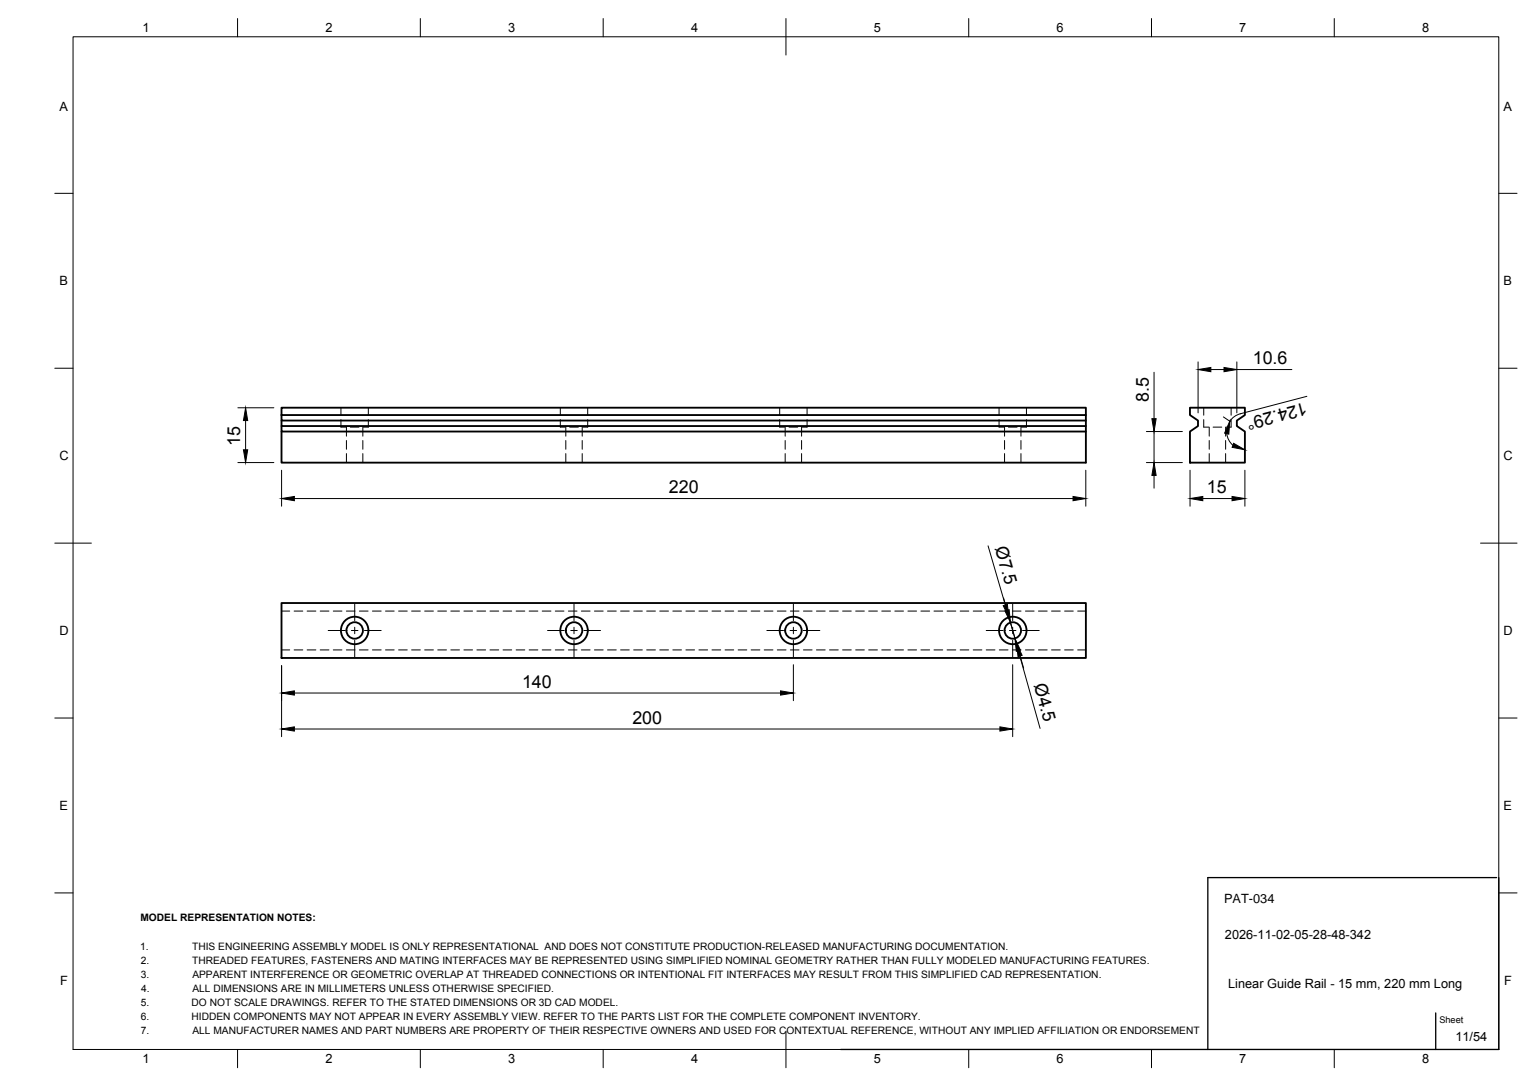
ISO-10303-21;
HEADER;
/* Generated by software containing ST-Developer
 * from STEP Tools, Inc. (www.steptools.com) 
 */

FILE_DESCRIPTION(
/* description */ ('Fatigue rig crank-slider'),
/* implementation_level */ '2;1');

FILE_NAME(
/* name */ 'Linear Guide Rail - 15 mm, 220 mm Long.step',
/* time_stamp */ '2026-10-28T03:24:50-07:00',
/* author */ (''),
/* organization */ (''),
/* preprocessor_version */ 'ST-DEVELOPER v20.2',
/* originating_system */ 'Autodesk Translation Framework v15.17.0.0',
/* authorisation */ '');

FILE_SCHEMA (('AUTOMOTIVE_DESIGN { 1 0 10303 214 3 1 1 }'));
ENDSEC;

DATA;
#10=MECHANICAL_DESIGN_GEOMETRIC_PRESENTATION_REPRESENTATION('',(#602),#16911);
#501=SHAPE_REPRESENTATION_RELATIONSHIP('SRR','None',#17141,#551);
#551=ADVANCED_BREP_SHAPE_REPRESENTATION('',(#660),#16870);
#602=STYLED_ITEM('',(#17480),#660);
#660=MANIFOLD_SOLID_BREP('Body1',#8894);
#808=FACE_BOUND('',#2027,.T.);
#809=FACE_BOUND('',#2030,.T.);
#810=FACE_BOUND('',#2033,.T.);
#811=FACE_BOUND('',#2036,.T.);
#812=FACE_BOUND('',#2046,.T.);
#813=FACE_BOUND('',#2047,.T.);
#814=FACE_BOUND('',#2048,.T.);
#815=FACE_BOUND('',#2049,.T.);
#816=FACE_BOUND('',#2056,.T.);
#817=FACE_BOUND('',#2057,.T.);
#818=FACE_BOUND('',#2058,.T.);
#819=FACE_BOUND('',#2059,.T.);
#998=PLANE('',#9834);
#999=PLANE('',#9839);
#1000=PLANE('',#9844);
#1001=PLANE('',#9849);
#1002=PLANE('',#9859);
#1003=PLANE('',#9860);
#1004=PLANE('',#9861);
#1005=PLANE('',#9862);
#1006=PLANE('',#9863);
#1007=PLANE('',#9864);
#1008=PLANE('',#9865);
#1009=PLANE('',#9866);
#1010=PLANE('',#9867);
#1011=PLANE('',#9868);
#1012=PLANE('',#9869);
#1013=PLANE('',#9870);
#1014=PLANE('',#9871);
#1015=PLANE('',#9872);
#1394=FACE_OUTER_BOUND('',#2025,.T.);
#1395=FACE_OUTER_BOUND('',#2026,.T.);
#1396=FACE_OUTER_BOUND('',#2028,.T.);
#1397=FACE_OUTER_BOUND('',#2029,.T.);
#1398=FACE_OUTER_BOUND('',#2031,.T.);
#1399=FACE_OUTER_BOUND('',#2032,.T.);
#1400=FACE_OUTER_BOUND('',#2034,.T.);
#1401=FACE_OUTER_BOUND('',#2035,.T.);
#1402=FACE_OUTER_BOUND('',#2037,.T.);
#1403=FACE_OUTER_BOUND('',#2038,.T.);
#1404=FACE_OUTER_BOUND('',#2039,.T.);
#1405=FACE_OUTER_BOUND('',#2040,.T.);
#1406=FACE_OUTER_BOUND('',#2041,.T.);
#1407=FACE_OUTER_BOUND('',#2042,.T.);
#1408=FACE_OUTER_BOUND('',#2043,.T.);
#1409=FACE_OUTER_BOUND('',#2044,.T.);
#1410=FACE_OUTER_BOUND('',#2045,.T.);
#1411=FACE_OUTER_BOUND('',#2050,.T.);
#1412=FACE_OUTER_BOUND('',#2051,.T.);
#1413=FACE_OUTER_BOUND('',#2052,.T.);
#1414=FACE_OUTER_BOUND('',#2053,.T.);
#1415=FACE_OUTER_BOUND('',#2054,.T.);
#1416=FACE_OUTER_BOUND('',#2055,.T.);
#1417=FACE_OUTER_BOUND('',#2060,.T.);
#1418=FACE_OUTER_BOUND('',#2061,.T.);
#1419=FACE_OUTER_BOUND('',#2062,.T.);
#2025=EDGE_LOOP('',(#6736,#6737,#6738,#6739));
#2026=EDGE_LOOP('',(#6740));
#2027=EDGE_LOOP('',(#6741));
#2028=EDGE_LOOP('',(#6742,#6743,#6744,#6745));
#2029=EDGE_LOOP('',(#6746));
#2030=EDGE_LOOP('',(#6747));
#2031=EDGE_LOOP('',(#6748,#6749,#6750,#6751));
#2032=EDGE_LOOP('',(#6752));
#2033=EDGE_LOOP('',(#6753));
#2034=EDGE_LOOP('',(#6754,#6755,#6756,#6757));
#2035=EDGE_LOOP('',(#6758));
#2036=EDGE_LOOP('',(#6759));
#2037=EDGE_LOOP('',(#6760,#6761,#6762,#6763));
#2038=EDGE_LOOP('',(#6764,#6765,#6766,#6767));
#2039=EDGE_LOOP('',(#6768,#6769,#6770,#6771));
#2040=EDGE_LOOP('',(#6772,#6773,#6774,#6775));
#2041=EDGE_LOOP('',(#6776,#6777,#6778,#6779));
#2042=EDGE_LOOP('',(#6780,#6781,#6782,#6783));
#2043=EDGE_LOOP('',(#6784,#6785,#6786,#6787));
#2044=EDGE_LOOP('',(#6788,#6789,#6790,#6791));
#2045=EDGE_LOOP('',(#6792,#6793,#6794,#6795));
#2046=EDGE_LOOP('',(#6796));
#2047=EDGE_LOOP('',(#6797));
#2048=EDGE_LOOP('',(#6798));
#2049=EDGE_LOOP('',(#6799));
#2050=EDGE_LOOP('',(#6800,#6801,#6802,#6803));
#2051=EDGE_LOOP('',(#6804,#6805,#6806,#6807));
#2052=EDGE_LOOP('',(#6808,#6809,#6810,#6811));
#2053=EDGE_LOOP('',(#6812,#6813,#6814,#6815));
#2054=EDGE_LOOP('',(#6816,#6817,#6818,#6819));
#2055=EDGE_LOOP('',(#6820,#6821,#6822,#6823));
#2056=EDGE_LOOP('',(#6824));
#2057=EDGE_LOOP('',(#6825));
#2058=EDGE_LOOP('',(#6826));
#2059=EDGE_LOOP('',(#6827));
#2060=EDGE_LOOP('',(#6828,#6829,#6830,#6831));
#2061=EDGE_LOOP('',(#6832,#6833,#6834,#6835,#6836,#6837,#6838,#6839,#6840,
#6841,#6842,#6843));
#2062=EDGE_LOOP('',(#6844,#6845,#6846,#6847,#6848,#6849,#6850,#6851,#6852,
#6853,#6854,#6855));
#2665=LINE('',#14590,#3311);
#2666=LINE('',#14599,#3312);
#2667=LINE('',#14608,#3313);
#2668=LINE('',#14617,#3314);
#2669=LINE('',#14625,#3315);
#2670=LINE('',#14629,#3316);
#2671=LINE('',#14633,#3317);
#2672=LINE('',#14637,#3318);
#2673=LINE('',#14641,#3319);
#2674=LINE('',#14643,#3320);
#2675=LINE('',#14645,#3321);
#2676=LINE('',#14646,#3322);
#2677=LINE('',#14649,#3323);
#2678=LINE('',#14651,#3324);
#2679=LINE('',#14652,#3325);
#2680=LINE('',#14655,#3326);
#2681=LINE('',#14657,#3327);
#2682=LINE('',#14658,#3328);
#2683=LINE('',#14661,#3329);
#2684=LINE('',#14663,#3330);
#2685=LINE('',#14664,#3331);
#2686=LINE('',#14667,#3332);
#2687=LINE('',#14669,#3333);
#2688=LINE('',#14670,#3334);
#2689=LINE('',#14673,#3335);
#2690=LINE('',#14675,#3336);
#2691=LINE('',#14676,#3337);
#2692=LINE('',#14679,#3338);
#2693=LINE('',#14681,#3339);
#2694=LINE('',#14682,#3340);
#2695=LINE('',#14685,#3341);
#2696=LINE('',#14687,#3342);
#2697=LINE('',#14688,#3343);
#2698=LINE('',#14691,#3344);
#2699=LINE('',#14693,#3345);
#2700=LINE('',#14694,#3346);
#2701=LINE('',#14697,#3347);
#2702=LINE('',#14699,#3348);
#2703=LINE('',#14700,#3349);
#2704=LINE('',#14703,#3350);
#2705=LINE('',#14705,#3351);
#2706=LINE('',#14706,#3352);
#2707=LINE('',#14708,#3353);
#2708=LINE('',#14709,#3354);
#3311=VECTOR('',#11451,0.375);
#3312=VECTOR('',#11462,0.375);
#3313=VECTOR('',#11473,0.375);
#3314=VECTOR('',#11484,0.375);
#3315=VECTOR('',#11495,0.225);
#3316=VECTOR('',#11500,0.225);
#3317=VECTOR('',#11505,0.225);
#3318=VECTOR('',#11510,0.225000000000001);
#3319=VECTOR('',#11513,1.);
#3320=VECTOR('',#11514,1.);
#3321=VECTOR('',#11515,1.);
#3322=VECTOR('',#11516,1.);
#3323=VECTOR('',#11519,1.);
#3324=VECTOR('',#11520,1.);
#3325=VECTOR('',#11521,1.);
#3326=VECTOR('',#11524,1.);
#3327=VECTOR('',#11525,1.);
#3328=VECTOR('',#11526,1.);
#3329=VECTOR('',#11529,1.);
#3330=VECTOR('',#11530,1.);
#3331=VECTOR('',#11531,1.);
#3332=VECTOR('',#11534,1.);
#3333=VECTOR('',#11535,1.);
#3334=VECTOR('',#11536,1.);
#3335=VECTOR('',#11539,1.);
#3336=VECTOR('',#11540,1.);
#3337=VECTOR('',#11541,1.);
#3338=VECTOR('',#11544,1.);
#3339=VECTOR('',#11545,1.);
#3340=VECTOR('',#11546,1.);
#3341=VECTOR('',#11549,1.);
#3342=VECTOR('',#11550,1.);
#3343=VECTOR('',#11551,1.);
#3344=VECTOR('',#11554,1.);
#3345=VECTOR('',#11555,1.);
#3346=VECTOR('',#11556,1.);
#3347=VECTOR('',#11559,1.);
#3348=VECTOR('',#11560,1.);
#3349=VECTOR('',#11561,1.);
#3350=VECTOR('',#11564,1.);
#3351=VECTOR('',#11565,1.);
#3352=VECTOR('',#11566,1.);
#3353=VECTOR('',#11569,1.);
#3354=VECTOR('',#11570,1.);
#3893=CIRCLE('',#9832,0.375);
#3894=CIRCLE('',#9833,0.375);
#3895=CIRCLE('',#9835,0.225);
#3896=CIRCLE('',#9837,0.375);
#3897=CIRCLE('',#9838,0.375);
#3898=CIRCLE('',#9840,0.225);
#3899=CIRCLE('',#9842,0.375);
#3900=CIRCLE('',#9843,0.375);
#3901=CIRCLE('',#9845,0.225);
#3902=CIRCLE('',#9847,0.375);
#3903=CIRCLE('',#9848,0.375);
#3904=CIRCLE('',#9850,0.225000000000001);
#3905=CIRCLE('',#9852,0.225);
#3906=CIRCLE('',#9854,0.225);
#3907=CIRCLE('',#9856,0.225);
#3908=CIRCLE('',#9858,0.225000000000001);
#4405=VERTEX_POINT('',#14587);
#4406=VERTEX_POINT('',#14589);
#4407=VERTEX_POINT('',#14593);
#4408=VERTEX_POINT('',#14596);
#4409=VERTEX_POINT('',#14598);
#4410=VERTEX_POINT('',#14602);
#4411=VERTEX_POINT('',#14605);
#4412=VERTEX_POINT('',#14607);
#4413=VERTEX_POINT('',#14611);
#4414=VERTEX_POINT('',#14614);
#4415=VERTEX_POINT('',#14616);
#4416=VERTEX_POINT('',#14620);
#4417=VERTEX_POINT('',#14623);
#4418=VERTEX_POINT('',#14627);
#4419=VERTEX_POINT('',#14631);
#4420=VERTEX_POINT('',#14635);
#4421=VERTEX_POINT('',#14639);
#4422=VERTEX_POINT('',#14640);
#4423=VERTEX_POINT('',#14642);
#4424=VERTEX_POINT('',#14644);
#4425=VERTEX_POINT('',#14648);
#4426=VERTEX_POINT('',#14650);
#4427=VERTEX_POINT('',#14654);
#4428=VERTEX_POINT('',#14656);
#4429=VERTEX_POINT('',#14660);
#4430=VERTEX_POINT('',#14662);
#4431=VERTEX_POINT('',#14666);
#4432=VERTEX_POINT('',#14668);
#4433=VERTEX_POINT('',#14672);
#4434=VERTEX_POINT('',#14674);
#4435=VERTEX_POINT('',#14678);
#4436=VERTEX_POINT('',#14680);
#4437=VERTEX_POINT('',#14684);
#4438=VERTEX_POINT('',#14686);
#4439=VERTEX_POINT('',#14690);
#4440=VERTEX_POINT('',#14692);
#4441=VERTEX_POINT('',#14696);
#4442=VERTEX_POINT('',#14698);
#4443=VERTEX_POINT('',#14702);
#4444=VERTEX_POINT('',#14704);
#5266=EDGE_CURVE('',#4405,#4405,#3893,.T.);
#5267=EDGE_CURVE('',#4405,#4406,#2665,.T.);
#5268=EDGE_CURVE('',#4406,#4406,#3894,.T.);
#5269=EDGE_CURVE('',#4407,#4407,#3895,.T.);
#5270=EDGE_CURVE('',#4408,#4408,#3896,.T.);
#5271=EDGE_CURVE('',#4408,#4409,#2666,.T.);
#5272=EDGE_CURVE('',#4409,#4409,#3897,.T.);
#5273=EDGE_CURVE('',#4410,#4410,#3898,.T.);
#5274=EDGE_CURVE('',#4411,#4411,#3899,.T.);
#5275=EDGE_CURVE('',#4411,#4412,#2667,.T.);
#5276=EDGE_CURVE('',#4412,#4412,#3900,.T.);
#5277=EDGE_CURVE('',#4413,#4413,#3901,.T.);
#5278=EDGE_CURVE('',#4414,#4414,#3902,.T.);
#5279=EDGE_CURVE('',#4414,#4415,#2668,.T.);
#5280=EDGE_CURVE('',#4415,#4415,#3903,.T.);
#5281=EDGE_CURVE('',#4416,#4416,#3904,.T.);
#5282=EDGE_CURVE('',#4417,#4417,#3905,.T.);
#5283=EDGE_CURVE('',#4417,#4407,#2669,.T.);
#5284=EDGE_CURVE('',#4418,#4418,#3906,.T.);
#5285=EDGE_CURVE('',#4418,#4410,#2670,.T.);
#5286=EDGE_CURVE('',#4419,#4419,#3907,.T.);
#5287=EDGE_CURVE('',#4419,#4413,#2671,.T.);
#5288=EDGE_CURVE('',#4420,#4420,#3908,.T.);
#5289=EDGE_CURVE('',#4420,#4416,#2672,.T.);
#5290=EDGE_CURVE('',#4421,#4422,#2673,.T.);
#5291=EDGE_CURVE('',#4422,#4423,#2674,.T.);
#5292=EDGE_CURVE('',#4424,#4423,#2675,.T.);
#5293=EDGE_CURVE('',#4421,#4424,#2676,.T.);
#5294=EDGE_CURVE('',#4425,#4421,#2677,.T.);
#5295=EDGE_CURVE('',#4426,#4424,#2678,.T.);
#5296=EDGE_CURVE('',#4425,#4426,#2679,.T.);
#5297=EDGE_CURVE('',#4427,#4425,#2680,.T.);
#5298=EDGE_CURVE('',#4428,#4426,#2681,.T.);
#5299=EDGE_CURVE('',#4427,#4428,#2682,.T.);
#5300=EDGE_CURVE('',#4429,#4427,#2683,.T.);
#5301=EDGE_CURVE('',#4430,#4428,#2684,.T.);
#5302=EDGE_CURVE('',#4429,#4430,#2685,.T.);
#5303=EDGE_CURVE('',#4431,#4429,#2686,.T.);
#5304=EDGE_CURVE('',#4432,#4430,#2687,.T.);
#5305=EDGE_CURVE('',#4431,#4432,#2688,.T.);
#5306=EDGE_CURVE('',#4433,#4431,#2689,.T.);
#5307=EDGE_CURVE('',#4434,#4432,#2690,.T.);
#5308=EDGE_CURVE('',#4433,#4434,#2691,.T.);
#5309=EDGE_CURVE('',#4435,#4433,#2692,.T.);
#5310=EDGE_CURVE('',#4436,#4434,#2693,.T.);
#5311=EDGE_CURVE('',#4435,#4436,#2694,.T.);
#5312=EDGE_CURVE('',#4437,#4435,#2695,.T.);
#5313=EDGE_CURVE('',#4438,#4436,#2696,.T.);
#5314=EDGE_CURVE('',#4437,#4438,#2697,.T.);
#5315=EDGE_CURVE('',#4439,#4437,#2698,.T.);
#5316=EDGE_CURVE('',#4440,#4438,#2699,.T.);
#5317=EDGE_CURVE('',#4439,#4440,#2700,.T.);
#5318=EDGE_CURVE('',#4441,#4439,#2701,.T.);
#5319=EDGE_CURVE('',#4442,#4440,#2702,.T.);
#5320=EDGE_CURVE('',#4441,#4442,#2703,.T.);
#5321=EDGE_CURVE('',#4443,#4441,#2704,.T.);
#5322=EDGE_CURVE('',#4444,#4442,#2705,.T.);
#5323=EDGE_CURVE('',#4443,#4444,#2706,.T.);
#5324=EDGE_CURVE('',#4422,#4443,#2707,.T.);
#5325=EDGE_CURVE('',#4423,#4444,#2708,.T.);
#6736=ORIENTED_EDGE('',*,*,#5266,.F.);
#6737=ORIENTED_EDGE('',*,*,#5267,.T.);
#6738=ORIENTED_EDGE('',*,*,#5268,.F.);
#6739=ORIENTED_EDGE('',*,*,#5267,.F.);
#6740=ORIENTED_EDGE('',*,*,#5266,.T.);
#6741=ORIENTED_EDGE('',*,*,#5269,.F.);
#6742=ORIENTED_EDGE('',*,*,#5270,.F.);
#6743=ORIENTED_EDGE('',*,*,#5271,.T.);
#6744=ORIENTED_EDGE('',*,*,#5272,.F.);
#6745=ORIENTED_EDGE('',*,*,#5271,.F.);
#6746=ORIENTED_EDGE('',*,*,#5270,.T.);
#6747=ORIENTED_EDGE('',*,*,#5273,.F.);
#6748=ORIENTED_EDGE('',*,*,#5274,.F.);
#6749=ORIENTED_EDGE('',*,*,#5275,.T.);
#6750=ORIENTED_EDGE('',*,*,#5276,.F.);
#6751=ORIENTED_EDGE('',*,*,#5275,.F.);
#6752=ORIENTED_EDGE('',*,*,#5274,.T.);
#6753=ORIENTED_EDGE('',*,*,#5277,.F.);
#6754=ORIENTED_EDGE('',*,*,#5278,.F.);
#6755=ORIENTED_EDGE('',*,*,#5279,.T.);
#6756=ORIENTED_EDGE('',*,*,#5280,.F.);
#6757=ORIENTED_EDGE('',*,*,#5279,.F.);
#6758=ORIENTED_EDGE('',*,*,#5278,.T.);
#6759=ORIENTED_EDGE('',*,*,#5281,.F.);
#6760=ORIENTED_EDGE('',*,*,#5282,.F.);
#6761=ORIENTED_EDGE('',*,*,#5283,.T.);
#6762=ORIENTED_EDGE('',*,*,#5269,.T.);
#6763=ORIENTED_EDGE('',*,*,#5283,.F.);
#6764=ORIENTED_EDGE('',*,*,#5284,.F.);
#6765=ORIENTED_EDGE('',*,*,#5285,.T.);
#6766=ORIENTED_EDGE('',*,*,#5273,.T.);
#6767=ORIENTED_EDGE('',*,*,#5285,.F.);
#6768=ORIENTED_EDGE('',*,*,#5286,.F.);
#6769=ORIENTED_EDGE('',*,*,#5287,.T.);
#6770=ORIENTED_EDGE('',*,*,#5277,.T.);
#6771=ORIENTED_EDGE('',*,*,#5287,.F.);
#6772=ORIENTED_EDGE('',*,*,#5288,.F.);
#6773=ORIENTED_EDGE('',*,*,#5289,.T.);
#6774=ORIENTED_EDGE('',*,*,#5281,.T.);
#6775=ORIENTED_EDGE('',*,*,#5289,.F.);
#6776=ORIENTED_EDGE('',*,*,#5290,.T.);
#6777=ORIENTED_EDGE('',*,*,#5291,.T.);
#6778=ORIENTED_EDGE('',*,*,#5292,.F.);
#6779=ORIENTED_EDGE('',*,*,#5293,.F.);
#6780=ORIENTED_EDGE('',*,*,#5294,.T.);
#6781=ORIENTED_EDGE('',*,*,#5293,.T.);
#6782=ORIENTED_EDGE('',*,*,#5295,.F.);
#6783=ORIENTED_EDGE('',*,*,#5296,.F.);
#6784=ORIENTED_EDGE('',*,*,#5297,.T.);
#6785=ORIENTED_EDGE('',*,*,#5296,.T.);
#6786=ORIENTED_EDGE('',*,*,#5298,.F.);
#6787=ORIENTED_EDGE('',*,*,#5299,.F.);
#6788=ORIENTED_EDGE('',*,*,#5300,.T.);
#6789=ORIENTED_EDGE('',*,*,#5299,.T.);
#6790=ORIENTED_EDGE('',*,*,#5301,.F.);
#6791=ORIENTED_EDGE('',*,*,#5302,.F.);
#6792=ORIENTED_EDGE('',*,*,#5303,.T.);
#6793=ORIENTED_EDGE('',*,*,#5302,.T.);
#6794=ORIENTED_EDGE('',*,*,#5304,.F.);
#6795=ORIENTED_EDGE('',*,*,#5305,.F.);
#6796=ORIENTED_EDGE('',*,*,#5280,.T.);
#6797=ORIENTED_EDGE('',*,*,#5276,.T.);
#6798=ORIENTED_EDGE('',*,*,#5272,.T.);
#6799=ORIENTED_EDGE('',*,*,#5268,.T.);
#6800=ORIENTED_EDGE('',*,*,#5306,.T.);
#6801=ORIENTED_EDGE('',*,*,#5305,.T.);
#6802=ORIENTED_EDGE('',*,*,#5307,.F.);
#6803=ORIENTED_EDGE('',*,*,#5308,.F.);
#6804=ORIENTED_EDGE('',*,*,#5309,.T.);
#6805=ORIENTED_EDGE('',*,*,#5308,.T.);
#6806=ORIENTED_EDGE('',*,*,#5310,.F.);
#6807=ORIENTED_EDGE('',*,*,#5311,.F.);
#6808=ORIENTED_EDGE('',*,*,#5312,.T.);
#6809=ORIENTED_EDGE('',*,*,#5311,.T.);
#6810=ORIENTED_EDGE('',*,*,#5313,.F.);
#6811=ORIENTED_EDGE('',*,*,#5314,.F.);
#6812=ORIENTED_EDGE('',*,*,#5315,.T.);
#6813=ORIENTED_EDGE('',*,*,#5314,.T.);
#6814=ORIENTED_EDGE('',*,*,#5316,.F.);
#6815=ORIENTED_EDGE('',*,*,#5317,.F.);
#6816=ORIENTED_EDGE('',*,*,#5318,.T.);
#6817=ORIENTED_EDGE('',*,*,#5317,.T.);
#6818=ORIENTED_EDGE('',*,*,#5319,.F.);
#6819=ORIENTED_EDGE('',*,*,#5320,.F.);
#6820=ORIENTED_EDGE('',*,*,#5321,.T.);
#6821=ORIENTED_EDGE('',*,*,#5320,.T.);
#6822=ORIENTED_EDGE('',*,*,#5322,.F.);
#6823=ORIENTED_EDGE('',*,*,#5323,.F.);
#6824=ORIENTED_EDGE('',*,*,#5282,.T.);
#6825=ORIENTED_EDGE('',*,*,#5284,.T.);
#6826=ORIENTED_EDGE('',*,*,#5286,.T.);
#6827=ORIENTED_EDGE('',*,*,#5288,.T.);
#6828=ORIENTED_EDGE('',*,*,#5324,.T.);
#6829=ORIENTED_EDGE('',*,*,#5323,.T.);
#6830=ORIENTED_EDGE('',*,*,#5325,.F.);
#6831=ORIENTED_EDGE('',*,*,#5291,.F.);
#6832=ORIENTED_EDGE('',*,*,#5325,.T.);
#6833=ORIENTED_EDGE('',*,*,#5322,.T.);
#6834=ORIENTED_EDGE('',*,*,#5319,.T.);
#6835=ORIENTED_EDGE('',*,*,#5316,.T.);
#6836=ORIENTED_EDGE('',*,*,#5313,.T.);
#6837=ORIENTED_EDGE('',*,*,#5310,.T.);
#6838=ORIENTED_EDGE('',*,*,#5307,.T.);
#6839=ORIENTED_EDGE('',*,*,#5304,.T.);
#6840=ORIENTED_EDGE('',*,*,#5301,.T.);
#6841=ORIENTED_EDGE('',*,*,#5298,.T.);
#6842=ORIENTED_EDGE('',*,*,#5295,.T.);
#6843=ORIENTED_EDGE('',*,*,#5292,.T.);
#6844=ORIENTED_EDGE('',*,*,#5324,.F.);
#6845=ORIENTED_EDGE('',*,*,#5290,.F.);
#6846=ORIENTED_EDGE('',*,*,#5294,.F.);
#6847=ORIENTED_EDGE('',*,*,#5297,.F.);
#6848=ORIENTED_EDGE('',*,*,#5300,.F.);
#6849=ORIENTED_EDGE('',*,*,#5303,.F.);
#6850=ORIENTED_EDGE('',*,*,#5306,.F.);
#6851=ORIENTED_EDGE('',*,*,#5309,.F.);
#6852=ORIENTED_EDGE('',*,*,#5312,.F.);
#6853=ORIENTED_EDGE('',*,*,#5315,.F.);
#6854=ORIENTED_EDGE('',*,*,#5318,.F.);
#6855=ORIENTED_EDGE('',*,*,#5321,.F.);
#8267=CYLINDRICAL_SURFACE('',#9831,0.375);
#8268=CYLINDRICAL_SURFACE('',#9836,0.375);
#8269=CYLINDRICAL_SURFACE('',#9841,0.375);
#8270=CYLINDRICAL_SURFACE('',#9846,0.375);
#8271=CYLINDRICAL_SURFACE('',#9851,0.225);
#8272=CYLINDRICAL_SURFACE('',#9853,0.225);
#8273=CYLINDRICAL_SURFACE('',#9855,0.225);
#8274=CYLINDRICAL_SURFACE('',#9857,0.225000000000001);
#8532=ADVANCED_FACE('',(#1394),#8267,.F.);
#8533=ADVANCED_FACE('',(#1395,#808),#998,.T.);
#8534=ADVANCED_FACE('',(#1396),#8268,.F.);
#8535=ADVANCED_FACE('',(#1397,#809),#999,.T.);
#8536=ADVANCED_FACE('',(#1398),#8269,.F.);
#8537=ADVANCED_FACE('',(#1399,#810),#1000,.T.);
#8538=ADVANCED_FACE('',(#1400),#8270,.F.);
#8539=ADVANCED_FACE('',(#1401,#811),#1001,.T.);
#8540=ADVANCED_FACE('',(#1402),#8271,.F.);
#8541=ADVANCED_FACE('',(#1403),#8272,.F.);
#8542=ADVANCED_FACE('',(#1404),#8273,.F.);
#8543=ADVANCED_FACE('',(#1405),#8274,.F.);
#8544=ADVANCED_FACE('',(#1406),#1002,.T.);
#8545=ADVANCED_FACE('',(#1407),#1003,.T.);
#8546=ADVANCED_FACE('',(#1408),#1004,.T.);
#8547=ADVANCED_FACE('',(#1409),#1005,.T.);
#8548=ADVANCED_FACE('',(#1410,#812,#813,#814,#815),#1006,.T.);
#8549=ADVANCED_FACE('',(#1411),#1007,.T.);
#8550=ADVANCED_FACE('',(#1412),#1008,.T.);
#8551=ADVANCED_FACE('',(#1413),#1009,.T.);
#8552=ADVANCED_FACE('',(#1414),#1010,.T.);
#8553=ADVANCED_FACE('',(#1415),#1011,.T.);
#8554=ADVANCED_FACE('',(#1416,#816,#817,#818,#819),#1012,.T.);
#8555=ADVANCED_FACE('',(#1417),#1013,.T.);
#8556=ADVANCED_FACE('',(#1418),#1014,.T.);
#8557=ADVANCED_FACE('',(#1419),#1015,.F.);
#8894=CLOSED_SHELL('',(#8532,#8533,#8534,#8535,#8536,#8537,#8538,#8539,
#8540,#8541,#8542,#8543,#8544,#8545,#8546,#8547,#8548,#8549,#8550,#8551,
#8552,#8553,#8554,#8555,#8556,#8557));
#9830=AXIS2_PLACEMENT_3D('',#14585,#11445,#11446);
#9831=AXIS2_PLACEMENT_3D('',#14586,#11447,#11448);
#9832=AXIS2_PLACEMENT_3D('',#14588,#11449,#11450);
#9833=AXIS2_PLACEMENT_3D('',#14591,#11452,#11453);
#9834=AXIS2_PLACEMENT_3D('',#14592,#11454,#11455);
#9835=AXIS2_PLACEMENT_3D('',#14594,#11456,#11457);
#9836=AXIS2_PLACEMENT_3D('',#14595,#11458,#11459);
#9837=AXIS2_PLACEMENT_3D('',#14597,#11460,#11461);
#9838=AXIS2_PLACEMENT_3D('',#14600,#11463,#11464);
#9839=AXIS2_PLACEMENT_3D('',#14601,#11465,#11466);
#9840=AXIS2_PLACEMENT_3D('',#14603,#11467,#11468);
#9841=AXIS2_PLACEMENT_3D('',#14604,#11469,#11470);
#9842=AXIS2_PLACEMENT_3D('',#14606,#11471,#11472);
#9843=AXIS2_PLACEMENT_3D('',#14609,#11474,#11475);
#9844=AXIS2_PLACEMENT_3D('',#14610,#11476,#11477);
#9845=AXIS2_PLACEMENT_3D('',#14612,#11478,#11479);
#9846=AXIS2_PLACEMENT_3D('',#14613,#11480,#11481);
#9847=AXIS2_PLACEMENT_3D('',#14615,#11482,#11483);
#9848=AXIS2_PLACEMENT_3D('',#14618,#11485,#11486);
#9849=AXIS2_PLACEMENT_3D('',#14619,#11487,#11488);
#9850=AXIS2_PLACEMENT_3D('',#14621,#11489,#11490);
#9851=AXIS2_PLACEMENT_3D('',#14622,#11491,#11492);
#9852=AXIS2_PLACEMENT_3D('',#14624,#11493,#11494);
#9853=AXIS2_PLACEMENT_3D('',#14626,#11496,#11497);
#9854=AXIS2_PLACEMENT_3D('',#14628,#11498,#11499);
#9855=AXIS2_PLACEMENT_3D('',#14630,#11501,#11502);
#9856=AXIS2_PLACEMENT_3D('',#14632,#11503,#11504);
#9857=AXIS2_PLACEMENT_3D('',#14634,#11506,#11507);
#9858=AXIS2_PLACEMENT_3D('',#14636,#11508,#11509);
#9859=AXIS2_PLACEMENT_3D('',#14638,#11511,#11512);
#9860=AXIS2_PLACEMENT_3D('',#14647,#11517,#11518);
#9861=AXIS2_PLACEMENT_3D('',#14653,#11522,#11523);
#9862=AXIS2_PLACEMENT_3D('',#14659,#11527,#11528);
#9863=AXIS2_PLACEMENT_3D('',#14665,#11532,#11533);
#9864=AXIS2_PLACEMENT_3D('',#14671,#11537,#11538);
#9865=AXIS2_PLACEMENT_3D('',#14677,#11542,#11543);
#9866=AXIS2_PLACEMENT_3D('',#14683,#11547,#11548);
#9867=AXIS2_PLACEMENT_3D('',#14689,#11552,#11553);
#9868=AXIS2_PLACEMENT_3D('',#14695,#11557,#11558);
#9869=AXIS2_PLACEMENT_3D('',#14701,#11562,#11563);
#9870=AXIS2_PLACEMENT_3D('',#14707,#11567,#11568);
#9871=AXIS2_PLACEMENT_3D('',#14710,#11571,#11572);
#9872=AXIS2_PLACEMENT_3D('',#14711,#11573,#11574);
#11445=DIRECTION('axis',(0.,0.,1.));
#11446=DIRECTION('refdir',(1.,0.,0.));
#11447=DIRECTION('center_axis',(0.,0.,1.));
#11448=DIRECTION('ref_axis',(1.,0.,0.));
#11449=DIRECTION('center_axis',(0.,0.,1.));
#11450=DIRECTION('ref_axis',(1.,0.,0.));
#11451=DIRECTION('',(0.,0.,1.));
#11452=DIRECTION('center_axis',(0.,0.,-1.));
#11453=DIRECTION('ref_axis',(1.,0.,0.));
#11454=DIRECTION('center_axis',(0.,0.,1.));
#11455=DIRECTION('ref_axis',(1.,0.,0.));
#11456=DIRECTION('center_axis',(0.,0.,1.));
#11457=DIRECTION('ref_axis',(1.,0.,0.));
#11458=DIRECTION('center_axis',(0.,0.,1.));
#11459=DIRECTION('ref_axis',(1.,0.,0.));
#11460=DIRECTION('center_axis',(0.,0.,1.));
#11461=DIRECTION('ref_axis',(1.,0.,0.));
#11462=DIRECTION('',(0.,0.,1.));
#11463=DIRECTION('center_axis',(0.,0.,-1.));
#11464=DIRECTION('ref_axis',(1.,0.,0.));
#11465=DIRECTION('center_axis',(0.,0.,1.));
#11466=DIRECTION('ref_axis',(1.,0.,0.));
#11467=DIRECTION('center_axis',(0.,0.,1.));
#11468=DIRECTION('ref_axis',(1.,0.,0.));
#11469=DIRECTION('center_axis',(0.,0.,1.));
#11470=DIRECTION('ref_axis',(1.,0.,0.));
#11471=DIRECTION('center_axis',(0.,0.,1.));
#11472=DIRECTION('ref_axis',(1.,0.,0.));
#11473=DIRECTION('',(0.,0.,1.));
#11474=DIRECTION('center_axis',(0.,0.,-1.));
#11475=DIRECTION('ref_axis',(1.,0.,0.));
#11476=DIRECTION('center_axis',(0.,0.,1.));
#11477=DIRECTION('ref_axis',(1.,0.,0.));
#11478=DIRECTION('center_axis',(0.,0.,1.));
#11479=DIRECTION('ref_axis',(1.,0.,0.));
#11480=DIRECTION('center_axis',(0.,0.,1.));
#11481=DIRECTION('ref_axis',(1.,0.,0.));
#11482=DIRECTION('center_axis',(0.,0.,1.));
#11483=DIRECTION('ref_axis',(1.,0.,0.));
#11484=DIRECTION('',(0.,0.,1.));
#11485=DIRECTION('center_axis',(0.,0.,-1.));
#11486=DIRECTION('ref_axis',(1.,0.,0.));
#11487=DIRECTION('center_axis',(0.,0.,1.));
#11488=DIRECTION('ref_axis',(1.,0.,0.));
#11489=DIRECTION('center_axis',(0.,0.,1.));
#11490=DIRECTION('ref_axis',(1.,0.,0.));
#11491=DIRECTION('center_axis',(0.,0.,1.));
#11492=DIRECTION('ref_axis',(1.,0.,0.));
#11493=DIRECTION('center_axis',(0.,0.,1.));
#11494=DIRECTION('ref_axis',(1.,0.,0.));
#11495=DIRECTION('',(0.,0.,1.));
#11496=DIRECTION('center_axis',(0.,0.,1.));
#11497=DIRECTION('ref_axis',(1.,0.,0.));
#11498=DIRECTION('center_axis',(0.,0.,1.));
#11499=DIRECTION('ref_axis',(1.,0.,0.));
#11500=DIRECTION('',(0.,0.,1.));
#11501=DIRECTION('center_axis',(0.,0.,1.));
#11502=DIRECTION('ref_axis',(1.,0.,0.));
#11503=DIRECTION('center_axis',(0.,0.,1.));
#11504=DIRECTION('ref_axis',(1.,0.,0.));
#11505=DIRECTION('',(0.,0.,1.));
#11506=DIRECTION('center_axis',(0.,0.,1.));
#11507=DIRECTION('ref_axis',(1.,0.,0.));
#11508=DIRECTION('center_axis',(0.,0.,1.));
#11509=DIRECTION('ref_axis',(1.,0.,0.));
#11510=DIRECTION('',(0.,0.,1.));
#11511=DIRECTION('center_axis',(0.,-0.56333682464151,0.826227342807548));
#11512=DIRECTION('ref_axis',(0.,-0.826227342807548,-0.56333682464151));
#11513=DIRECTION('',(0.,-0.826227342807548,-0.56333682464151));
#11514=DIRECTION('',(1.,0.,0.));
#11515=DIRECTION('',(0.,-0.826227342807548,-0.56333682464151));
#11516=DIRECTION('',(1.,0.,0.));
#11517=DIRECTION('center_axis',(0.,-1.,0.));
#11518=DIRECTION('ref_axis',(0.,0.,-1.));
#11519=DIRECTION('',(0.,0.,-1.));
#11520=DIRECTION('',(0.,0.,-1.));
#11521=DIRECTION('',(1.,0.,0.));
#11522=DIRECTION('center_axis',(0.,-0.56333682464151,-0.826227342807548));
#11523=DIRECTION('ref_axis',(0.,0.826227342807548,-0.56333682464151));
#11524=DIRECTION('',(0.,0.826227342807548,-0.56333682464151));
#11525=DIRECTION('',(0.,0.826227342807548,-0.56333682464151));
#11526=DIRECTION('',(1.,0.,0.));
#11527=DIRECTION('center_axis',(0.,-1.,0.));
#11528=DIRECTION('ref_axis',(0.,0.,-1.));
#11529=DIRECTION('',(0.,0.,-1.));
#11530=DIRECTION('',(0.,0.,-1.));
#11531=DIRECTION('',(1.,0.,0.));
#11532=DIRECTION('center_axis',(0.,0.,1.));
#11533=DIRECTION('ref_axis',(0.,-1.,0.));
#11534=DIRECTION('',(0.,-1.,0.));
#11535=DIRECTION('',(0.,-1.,0.));
#11536=DIRECTION('',(1.,0.,0.));
#11537=DIRECTION('center_axis',(0.,1.,0.));
#11538=DIRECTION('ref_axis',(0.,0.,1.));
#11539=DIRECTION('',(0.,0.,1.));
#11540=DIRECTION('',(0.,0.,1.));
#11541=DIRECTION('',(1.,0.,0.));
#11542=DIRECTION('center_axis',(0.,0.56333682464151,-0.826227342807548));
#11543=DIRECTION('ref_axis',(0.,0.826227342807548,0.56333682464151));
#11544=DIRECTION('',(0.,0.826227342807548,0.56333682464151));
#11545=DIRECTION('',(0.,0.826227342807548,0.56333682464151));
#11546=DIRECTION('',(1.,0.,0.));
#11547=DIRECTION('center_axis',(0.,1.,0.));
#11548=DIRECTION('ref_axis',(0.,0.,1.));
#11549=DIRECTION('',(0.,0.,1.));
#11550=DIRECTION('',(0.,0.,1.));
#11551=DIRECTION('',(1.,0.,0.));
#11552=DIRECTION('center_axis',(0.,0.56333682464151,0.826227342807548));
#11553=DIRECTION('ref_axis',(0.,-0.826227342807548,0.56333682464151));
#11554=DIRECTION('',(0.,-0.826227342807548,0.56333682464151));
#11555=DIRECTION('',(0.,-0.826227342807548,0.56333682464151));
#11556=DIRECTION('',(1.,0.,0.));
#11557=DIRECTION('center_axis',(0.,1.,0.));
#11558=DIRECTION('ref_axis',(0.,0.,1.));
#11559=DIRECTION('',(0.,0.,1.));
#11560=DIRECTION('',(0.,0.,1.));
#11561=DIRECTION('',(1.,0.,0.));
#11562=DIRECTION('center_axis',(0.,0.,-1.));
#11563=DIRECTION('ref_axis',(0.,1.,0.));
#11564=DIRECTION('',(0.,1.,0.));
#11565=DIRECTION('',(0.,1.,0.));
#11566=DIRECTION('',(1.,0.,0.));
#11567=DIRECTION('center_axis',(0.,-1.,0.));
#11568=DIRECTION('ref_axis',(0.,0.,-1.));
#11569=DIRECTION('',(0.,0.,-1.));
#11570=DIRECTION('',(0.,0.,-1.));
#11571=DIRECTION('center_axis',(1.,0.,0.));
#11572=DIRECTION('ref_axis',(0.,0.,-1.));
#11573=DIRECTION('center_axis',(1.,0.,0.));
#11574=DIRECTION('ref_axis',(0.,0.,-1.));
#14585=CARTESIAN_POINT('',(0.,0.,0.));
#14586=CARTESIAN_POINT('Origin',(14.,0.,0.97));
#14587=CARTESIAN_POINT('',(13.625,-4.59242549680257E-17,0.97));
#14588=CARTESIAN_POINT('Origin',(14.,0.,0.97));
#14589=CARTESIAN_POINT('',(13.625,4.59242549680257E-17,1.5));
#14590=CARTESIAN_POINT('',(13.625,-4.59242549680257E-17,0.97));
#14591=CARTESIAN_POINT('Origin',(14.,0.,1.5));
#14592=CARTESIAN_POINT('Origin',(14.,0.,0.97));
#14593=CARTESIAN_POINT('',(13.775,-2.75545529808154E-17,0.97));
#14594=CARTESIAN_POINT('Origin',(14.,0.,0.97));
#14595=CARTESIAN_POINT('Origin',(8.,0.,0.97));
#14596=CARTESIAN_POINT('',(7.625,-4.59242549680257E-17,0.97));
#14597=CARTESIAN_POINT('Origin',(8.,0.,0.97));
#14598=CARTESIAN_POINT('',(7.625,4.59242549680257E-17,1.5));
#14599=CARTESIAN_POINT('',(7.625,-4.59242549680257E-17,0.97));
#14600=CARTESIAN_POINT('Origin',(8.,0.,1.5));
#14601=CARTESIAN_POINT('Origin',(8.,0.,0.97));
#14602=CARTESIAN_POINT('',(7.775,-2.75545529808154E-17,0.97));
#14603=CARTESIAN_POINT('Origin',(8.,0.,0.97));
#14604=CARTESIAN_POINT('Origin',(2.,0.,0.97));
#14605=CARTESIAN_POINT('',(1.625,-4.59242549680257E-17,0.97));
#14606=CARTESIAN_POINT('Origin',(2.,0.,0.97));
#14607=CARTESIAN_POINT('',(1.625,4.59242549680257E-17,1.5));
#14608=CARTESIAN_POINT('',(1.625,-4.59242549680257E-17,0.97));
#14609=CARTESIAN_POINT('Origin',(2.,0.,1.5));
#14610=CARTESIAN_POINT('Origin',(2.,0.,0.97));
#14611=CARTESIAN_POINT('',(1.775,-2.75545529808155E-17,0.97));
#14612=CARTESIAN_POINT('Origin',(2.,0.,0.97));
#14613=CARTESIAN_POINT('Origin',(20.,0.,0.97));
#14614=CARTESIAN_POINT('',(19.625,-4.59242549680257E-17,0.97));
#14615=CARTESIAN_POINT('Origin',(20.,0.,0.97));
#14616=CARTESIAN_POINT('',(19.625,4.59242549680257E-17,1.5));
#14617=CARTESIAN_POINT('',(19.625,-4.59242549680257E-17,0.97));
#14618=CARTESIAN_POINT('Origin',(20.,0.,1.5));
#14619=CARTESIAN_POINT('Origin',(20.,0.,0.97));
#14620=CARTESIAN_POINT('',(19.775,-2.75545529808156E-17,0.97));
#14621=CARTESIAN_POINT('Origin',(20.,0.,0.97));
#14622=CARTESIAN_POINT('Origin',(14.,0.,-0.1));
#14623=CARTESIAN_POINT('',(13.775,-2.75545529808154E-17,0.));
#14624=CARTESIAN_POINT('Origin',(14.,0.,0.));
#14625=CARTESIAN_POINT('',(13.775,-2.75545529808154E-17,-0.1));
#14626=CARTESIAN_POINT('Origin',(8.,0.,-0.1));
#14627=CARTESIAN_POINT('',(7.775,-2.75545529808154E-17,0.));
#14628=CARTESIAN_POINT('Origin',(8.,0.,0.));
#14629=CARTESIAN_POINT('',(7.775,-2.75545529808154E-17,-0.1));
#14630=CARTESIAN_POINT('Origin',(2.,0.,-0.1));
#14631=CARTESIAN_POINT('',(1.775,-2.75545529808155E-17,0.));
#14632=CARTESIAN_POINT('Origin',(2.,0.,0.));
#14633=CARTESIAN_POINT('',(1.775,-2.75545529808155E-17,-0.1));
#14634=CARTESIAN_POINT('Origin',(20.,0.,-0.1));
#14635=CARTESIAN_POINT('',(19.775,-2.75545529808156E-17,0.));
#14636=CARTESIAN_POINT('Origin',(20.,0.,0.));
#14637=CARTESIAN_POINT('',(19.775,-2.75545529808156E-17,-0.1));
#14638=CARTESIAN_POINT('Origin',(0.,-0.53,1.));
#14639=CARTESIAN_POINT('',(0.,-0.53,1.));
#14640=CARTESIAN_POINT('',(0.,-0.75,0.85));
#14641=CARTESIAN_POINT('',(0.,-0.53,1.));
#14642=CARTESIAN_POINT('',(22.,-0.75,0.85));
#14643=CARTESIAN_POINT('',(0.,-0.75,0.85));
#14644=CARTESIAN_POINT('',(22.,-0.53,1.));
#14645=CARTESIAN_POINT('',(22.,-0.53,1.));
#14646=CARTESIAN_POINT('',(0.,-0.53,1.));
#14647=CARTESIAN_POINT('Origin',(0.,-0.53,1.15));
#14648=CARTESIAN_POINT('',(0.,-0.53,1.15));
#14649=CARTESIAN_POINT('',(0.,-0.53,1.15));
#14650=CARTESIAN_POINT('',(22.,-0.53,1.15));
#14651=CARTESIAN_POINT('',(22.,-0.53,1.15));
#14652=CARTESIAN_POINT('',(0.,-0.53,1.15));
#14653=CARTESIAN_POINT('Origin',(0.,-0.75,1.3));
#14654=CARTESIAN_POINT('',(0.,-0.75,1.3));
#14655=CARTESIAN_POINT('',(0.,-0.75,1.3));
#14656=CARTESIAN_POINT('',(22.,-0.75,1.3));
#14657=CARTESIAN_POINT('',(22.,-0.75,1.3));
#14658=CARTESIAN_POINT('',(0.,-0.75,1.3));
#14659=CARTESIAN_POINT('Origin',(0.,-0.75,1.5));
#14660=CARTESIAN_POINT('',(0.,-0.75,1.5));
#14661=CARTESIAN_POINT('',(0.,-0.75,1.5));
#14662=CARTESIAN_POINT('',(22.,-0.75,1.5));
#14663=CARTESIAN_POINT('',(22.,-0.75,1.5));
#14664=CARTESIAN_POINT('',(0.,-0.75,1.5));
#14665=CARTESIAN_POINT('Origin',(0.,0.75,1.5));
#14666=CARTESIAN_POINT('',(0.,0.75,1.5));
#14667=CARTESIAN_POINT('',(0.,0.75,1.5));
#14668=CARTESIAN_POINT('',(22.,0.75,1.5));
#14669=CARTESIAN_POINT('',(22.,0.75,1.5));
#14670=CARTESIAN_POINT('',(0.,0.75,1.5));
#14671=CARTESIAN_POINT('Origin',(0.,0.75,1.3));
#14672=CARTESIAN_POINT('',(0.,0.75,1.3));
#14673=CARTESIAN_POINT('',(0.,0.75,1.3));
#14674=CARTESIAN_POINT('',(22.,0.75,1.3));
#14675=CARTESIAN_POINT('',(22.,0.75,1.3));
#14676=CARTESIAN_POINT('',(0.,0.75,1.3));
#14677=CARTESIAN_POINT('Origin',(0.,0.53,1.15));
#14678=CARTESIAN_POINT('',(0.,0.53,1.15));
#14679=CARTESIAN_POINT('',(0.,0.53,1.15));
#14680=CARTESIAN_POINT('',(22.,0.53,1.15));
#14681=CARTESIAN_POINT('',(22.,0.53,1.15));
#14682=CARTESIAN_POINT('',(0.,0.53,1.15));
#14683=CARTESIAN_POINT('Origin',(0.,0.53,1.));
#14684=CARTESIAN_POINT('',(0.,0.53,1.));
#14685=CARTESIAN_POINT('',(0.,0.53,1.));
#14686=CARTESIAN_POINT('',(22.,0.53,1.));
#14687=CARTESIAN_POINT('',(22.,0.53,1.));
#14688=CARTESIAN_POINT('',(0.,0.53,1.));
#14689=CARTESIAN_POINT('Origin',(0.,0.75,0.85));
#14690=CARTESIAN_POINT('',(0.,0.75,0.85));
#14691=CARTESIAN_POINT('',(0.,0.75,0.85));
#14692=CARTESIAN_POINT('',(22.,0.75,0.85));
#14693=CARTESIAN_POINT('',(22.,0.75,0.85));
#14694=CARTESIAN_POINT('',(0.,0.75,0.85));
#14695=CARTESIAN_POINT('Origin',(0.,0.75,0.));
#14696=CARTESIAN_POINT('',(0.,0.75,0.));
#14697=CARTESIAN_POINT('',(0.,0.75,0.));
#14698=CARTESIAN_POINT('',(22.,0.75,0.));
#14699=CARTESIAN_POINT('',(22.,0.75,0.));
#14700=CARTESIAN_POINT('',(0.,0.75,0.));
#14701=CARTESIAN_POINT('Origin',(0.,-0.75,0.));
#14702=CARTESIAN_POINT('',(0.,-0.75,0.));
#14703=CARTESIAN_POINT('',(0.,-0.75,0.));
#14704=CARTESIAN_POINT('',(22.,-0.75,0.));
#14705=CARTESIAN_POINT('',(22.,-0.75,0.));
#14706=CARTESIAN_POINT('',(0.,-0.75,0.));
#14707=CARTESIAN_POINT('Origin',(0.,-0.75,0.85));
#14708=CARTESIAN_POINT('',(0.,-0.75,0.85));
#14709=CARTESIAN_POINT('',(22.,-0.75,0.85));
#14710=CARTESIAN_POINT('Origin',(22.,0.,0.75));
#14711=CARTESIAN_POINT('Origin',(0.,0.,0.75));
#16811=UNCERTAINTY_MEASURE_WITH_UNIT(LENGTH_MEASURE(0.001),#16912,
'DISTANCE_ACCURACY_VALUE',
'Maximum model space distance between geometric entities at asserted c
onnectivities');
#16852=UNCERTAINTY_MEASURE_WITH_UNIT(LENGTH_MEASURE(0.001),#16912,
'DISTANCE_ACCURACY_VALUE',
'Maximum model space distance between geometric entities at asserted c
onnectivities');
#16870=(
GEOMETRIC_REPRESENTATION_CONTEXT(3)
GLOBAL_UNCERTAINTY_ASSIGNED_CONTEXT((#16811))
GLOBAL_UNIT_ASSIGNED_CONTEXT((#16912,#16914,#16915))
REPRESENTATION_CONTEXT('','3D')
);
#16911=(
GEOMETRIC_REPRESENTATION_CONTEXT(3)
GLOBAL_UNCERTAINTY_ASSIGNED_CONTEXT((#16852))
GLOBAL_UNIT_ASSIGNED_CONTEXT((#16912,#16914,#16915))
REPRESENTATION_CONTEXT('','3D')
);
#16912=(
LENGTH_UNIT()
NAMED_UNIT(*)
SI_UNIT(.CENTI.,.METRE.)
);
#16914=(
NAMED_UNIT(*)
PLANE_ANGLE_UNIT()
SI_UNIT($,.RADIAN.)
);
#16915=(
NAMED_UNIT(*)
SI_UNIT($,.STERADIAN.)
SOLID_ANGLE_UNIT()
);
#16933=SHAPE_DEFINITION_REPRESENTATION(#16993,#17141);
#16993=PRODUCT_DEFINITION_SHAPE('',$,#17200);
#17141=SHAPE_REPRESENTATION('',(#9830),#16870);
#17182=PRODUCT_DEFINITION_CONTEXT('part definition',#17358,'design');
#17200=PRODUCT_DEFINITION('Linear Guide Rail - 15 mm, 220 mm Long',
'Linear Guide Rail - 15 mm, 220 mm Long',#17258,#17182);
#17258=PRODUCT_DEFINITION_FORMATION('',$,#17377);
#17358=APPLICATION_CONTEXT(
'Core Data for Automotive Mechanical Design Process');
#17359=PRODUCT_CONTEXT('part definition',#17358,'mechanical');
#17377=PRODUCT('Linear Guide Rail - 15 mm, 220 mm Long',
'Linear Guide Rail - 15 mm, 220 mm Long',
'Linear Guide Rail - 15 mm, 220 mm Long',(#17359));
#17474=COLOUR_RGB('Sky Blue',0.24,0.69,0.87);
#17475=FILL_AREA_STYLE_COLOUR('',#17474);
#17476=FILL_AREA_STYLE('',(#17475));
#17477=SURFACE_STYLE_FILL_AREA(#17476);
#17478=SURFACE_SIDE_STYLE('',(#17477));
#17479=SURFACE_STYLE_USAGE(.BOTH.,#17478);
#17480=PRESENTATION_STYLE_ASSIGNMENT((#17479));
ENDSEC;
END-ISO-10303-21;
